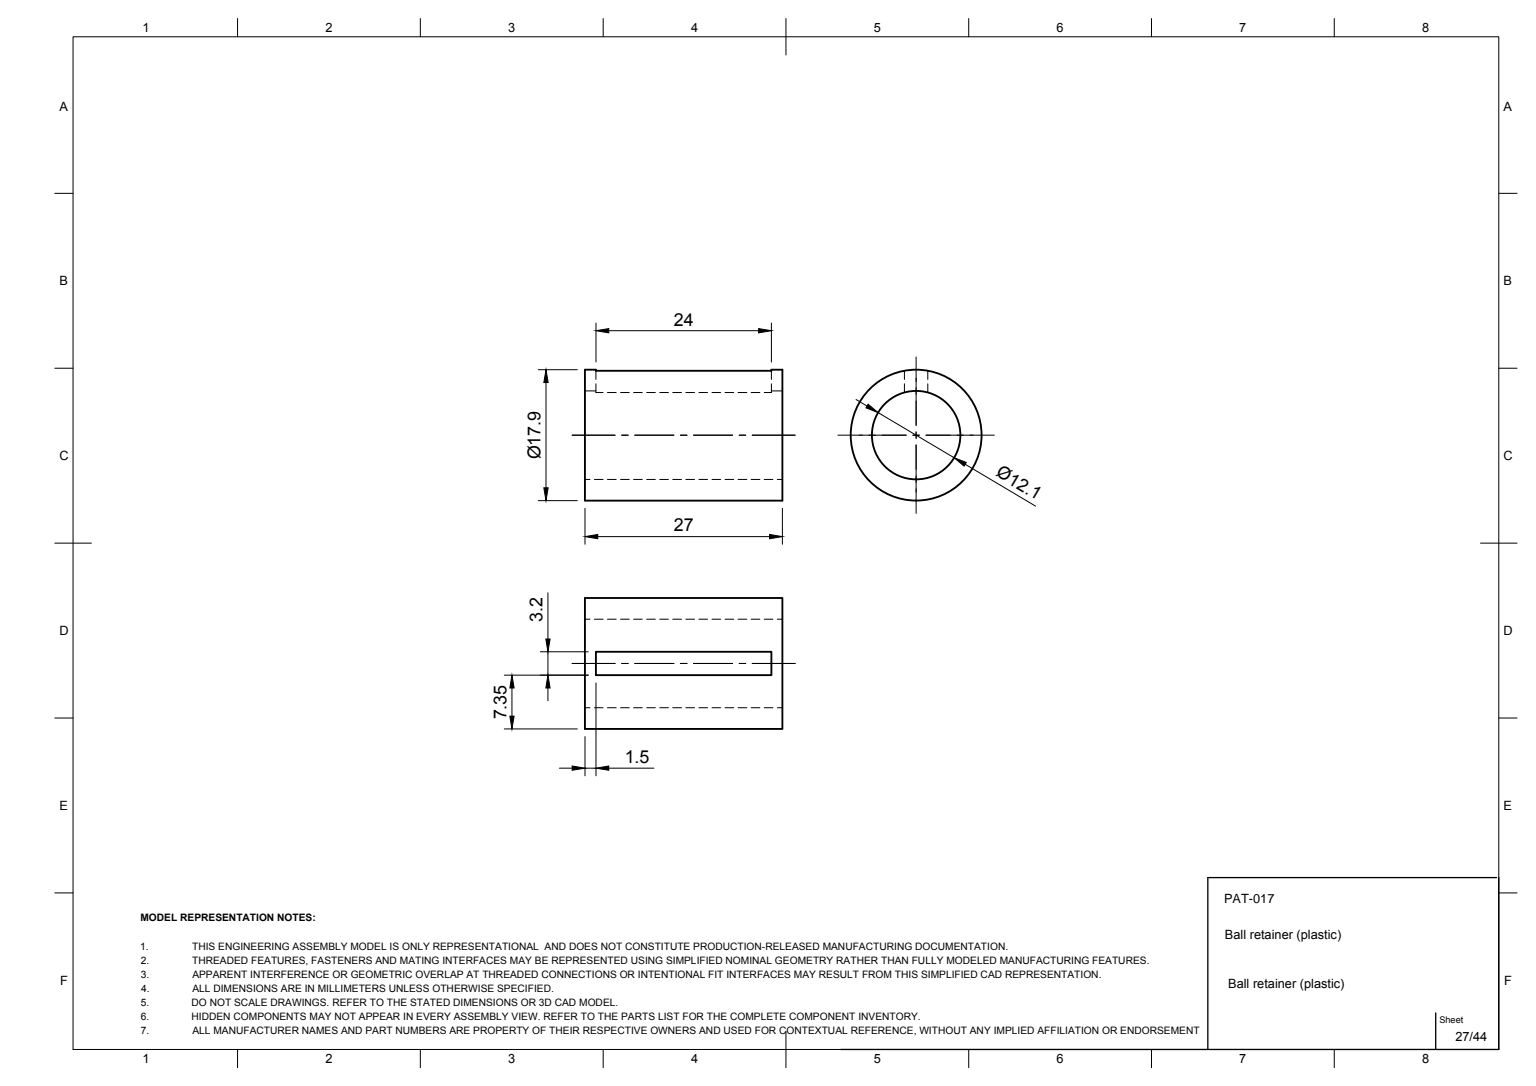
ISO-10303-21;
HEADER;
/* Generated by software containing ST-Developer
 * from STEP Tools, Inc. (www.steptools.com) 
 */

FILE_DESCRIPTION(
/* description */ ('Cam-and-follower valve demonstrator'),
/* implementation_level */ '2;1');

FILE_NAME(
/* name */ 'Ball retainer (plastic).step',
/* time_stamp */ '2026-10-28T03:25:17-07:00',
/* author */ (''),
/* organization */ (''),
/* preprocessor_version */ 'ST-DEVELOPER v20.2',
/* originating_system */ 'Autodesk Translation Framework v15.17.0.0',
/* authorisation */ '');

FILE_SCHEMA (('AUTOMOTIVE_DESIGN { 1 0 10303 214 3 1 1 }'));
ENDSEC;

DATA;
#10=MECHANICAL_DESIGN_GEOMETRIC_PRESENTATION_REPRESENTATION('',(#438),#12896);
#359=SHAPE_REPRESENTATION_RELATIONSHIP('SRR','None',#13077,#395);
#395=ADVANCED_BREP_SHAPE_REPRESENTATION('',(#480),#12877);
#438=STYLED_ITEM('',(#13323),#480);
#480=MANIFOLD_SOLID_BREP('Body1',#6206);
#621=FACE_BOUND('',#1823,.T.);
#622=FACE_BOUND('',#1825,.T.);
#623=FACE_BOUND('',#1827,.T.);
#624=FACE_BOUND('',#1829,.T.);
#882=CIRCLE('',#7103,0.895);
#883=CIRCLE('',#7104,0.605);
#884=CIRCLE('',#7107,0.895);
#885=CIRCLE('',#7108,0.605);
#886=CIRCLE('',#7111,0.895);
#887=CIRCLE('',#7112,0.605);
#888=CIRCLE('',#7114,0.895);
#889=CIRCLE('',#7116,0.605);
#1058=CYLINDRICAL_SURFACE('',#7113,0.895);
#1059=CYLINDRICAL_SURFACE('',#7117,0.605);
#1324=FACE_OUTER_BOUND('',#1818,.T.);
#1325=FACE_OUTER_BOUND('',#1819,.T.);
#1326=FACE_OUTER_BOUND('',#1820,.T.);
#1327=FACE_OUTER_BOUND('',#1821,.T.);
#1328=FACE_OUTER_BOUND('',#1822,.T.);
#1329=FACE_OUTER_BOUND('',#1824,.T.);
#1330=FACE_OUTER_BOUND('',#1826,.T.);
#1331=FACE_OUTER_BOUND('',#1828,.T.);
#1818=EDGE_LOOP('',(#5077,#5078,#5079,#5080));
#1819=EDGE_LOOP('',(#5081,#5082,#5083,#5084));
#1820=EDGE_LOOP('',(#5085,#5086,#5087,#5088));
#1821=EDGE_LOOP('',(#5089,#5090,#5091,#5092));
#1822=EDGE_LOOP('',(#5093));
#1823=EDGE_LOOP('',(#5094));
#1824=EDGE_LOOP('',(#5095,#5096,#5097,#5098));
#1825=EDGE_LOOP('',(#5099,#5100,#5101,#5102));
#1826=EDGE_LOOP('',(#5103));
#1827=EDGE_LOOP('',(#5104));
#1828=EDGE_LOOP('',(#5105,#5106,#5107,#5108));
#1829=EDGE_LOOP('',(#5109,#5110,#5111,#5112));
#2248=LINE('',#12164,#2670);
#2249=LINE('',#12167,#2671);
#2250=LINE('',#12170,#2672);
#2251=LINE('',#12172,#2673);
#2252=LINE('',#12173,#2674);
#2253=LINE('',#12179,#2675);
#2254=LINE('',#12181,#2676);
#2255=LINE('',#12182,#2677);
#2256=LINE('',#12191,#2678);
#2257=LINE('',#12196,#2679);
#2670=VECTOR('',#8631,1.);
#2671=VECTOR('',#8634,1.);
#2672=VECTOR('',#8637,1.);
#2673=VECTOR('',#8638,1.);
#2674=VECTOR('',#8639,1.);
#2675=VECTOR('',#8646,1.);
#2676=VECTOR('',#8649,1.);
#2677=VECTOR('',#8650,1.);
#2678=VECTOR('',#8661,0.895);
#2679=VECTOR('',#8668,0.605);
#3173=VERTEX_POINT('',#12160);
#3174=VERTEX_POINT('',#12161);
#3175=VERTEX_POINT('',#12163);
#3176=VERTEX_POINT('',#12165);
#3177=VERTEX_POINT('',#12169);
#3178=VERTEX_POINT('',#12171);
#3179=VERTEX_POINT('',#12175);
#3180=VERTEX_POINT('',#12177);
#3181=VERTEX_POINT('',#12184);
#3182=VERTEX_POINT('',#12186);
#3183=VERTEX_POINT('',#12189);
#3184=VERTEX_POINT('',#12193);
#3835=EDGE_CURVE('',#3173,#3174,#882,.T.);
#3836=EDGE_CURVE('',#3175,#3173,#2248,.T.);
#3837=EDGE_CURVE('',#3176,#3175,#883,.T.);
#3838=EDGE_CURVE('',#3174,#3176,#2249,.T.);
#3839=EDGE_CURVE('',#3174,#3177,#2250,.T.);
#3840=EDGE_CURVE('',#3178,#3176,#2251,.T.);
#3841=EDGE_CURVE('',#3178,#3177,#2252,.T.);
#3842=EDGE_CURVE('',#3177,#3179,#884,.T.);
#3843=EDGE_CURVE('',#3180,#3178,#885,.T.);
#3844=EDGE_CURVE('',#3179,#3180,#2253,.T.);
#3845=EDGE_CURVE('',#3179,#3173,#2254,.T.);
#3846=EDGE_CURVE('',#3175,#3180,#2255,.T.);
#3847=EDGE_CURVE('',#3181,#3181,#886,.T.);
#3848=EDGE_CURVE('',#3182,#3182,#887,.T.);
#3849=EDGE_CURVE('',#3183,#3183,#888,.T.);
#3850=EDGE_CURVE('',#3183,#3181,#2256,.T.);
#3851=EDGE_CURVE('',#3184,#3184,#889,.T.);
#3852=EDGE_CURVE('',#3184,#3182,#2257,.T.);
#5077=ORIENTED_EDGE('',*,*,#3835,.F.);
#5078=ORIENTED_EDGE('',*,*,#3836,.F.);
#5079=ORIENTED_EDGE('',*,*,#3837,.F.);
#5080=ORIENTED_EDGE('',*,*,#3838,.F.);
#5081=ORIENTED_EDGE('',*,*,#3839,.F.);
#5082=ORIENTED_EDGE('',*,*,#3838,.T.);
#5083=ORIENTED_EDGE('',*,*,#3840,.F.);
#5084=ORIENTED_EDGE('',*,*,#3841,.T.);
#5085=ORIENTED_EDGE('',*,*,#3842,.F.);
#5086=ORIENTED_EDGE('',*,*,#3841,.F.);
#5087=ORIENTED_EDGE('',*,*,#3843,.F.);
#5088=ORIENTED_EDGE('',*,*,#3844,.F.);
#5089=ORIENTED_EDGE('',*,*,#3845,.F.);
#5090=ORIENTED_EDGE('',*,*,#3844,.T.);
#5091=ORIENTED_EDGE('',*,*,#3846,.F.);
#5092=ORIENTED_EDGE('',*,*,#3836,.T.);
#5093=ORIENTED_EDGE('',*,*,#3847,.F.);
#5094=ORIENTED_EDGE('',*,*,#3848,.T.);
#5095=ORIENTED_EDGE('',*,*,#3849,.F.);
#5096=ORIENTED_EDGE('',*,*,#3850,.T.);
#5097=ORIENTED_EDGE('',*,*,#3847,.T.);
#5098=ORIENTED_EDGE('',*,*,#3850,.F.);
#5099=ORIENTED_EDGE('',*,*,#3842,.T.);
#5100=ORIENTED_EDGE('',*,*,#3845,.T.);
#5101=ORIENTED_EDGE('',*,*,#3835,.T.);
#5102=ORIENTED_EDGE('',*,*,#3839,.T.);
#5103=ORIENTED_EDGE('',*,*,#3849,.T.);
#5104=ORIENTED_EDGE('',*,*,#3851,.F.);
#5105=ORIENTED_EDGE('',*,*,#3851,.T.);
#5106=ORIENTED_EDGE('',*,*,#3852,.T.);
#5107=ORIENTED_EDGE('',*,*,#3848,.F.);
#5108=ORIENTED_EDGE('',*,*,#3852,.F.);
#5109=ORIENTED_EDGE('',*,*,#3843,.T.);
#5110=ORIENTED_EDGE('',*,*,#3840,.T.);
#5111=ORIENTED_EDGE('',*,*,#3837,.T.);
#5112=ORIENTED_EDGE('',*,*,#3846,.T.);
#5716=PLANE('',#7102);
#5717=PLANE('',#7105);
#5718=PLANE('',#7106);
#5719=PLANE('',#7109);
#5720=PLANE('',#7110);
#5721=PLANE('',#7115);
#6040=ADVANCED_FACE('',(#1324),#5716,.F.);
#6041=ADVANCED_FACE('',(#1325),#5717,.F.);
#6042=ADVANCED_FACE('',(#1326),#5718,.F.);
#6043=ADVANCED_FACE('',(#1327),#5719,.F.);
#6044=ADVANCED_FACE('',(#1328,#621),#5720,.T.);
#6045=ADVANCED_FACE('',(#1329,#622),#1058,.T.);
#6046=ADVANCED_FACE('',(#1330,#623),#5721,.T.);
#6047=ADVANCED_FACE('',(#1331,#624),#1059,.F.);
#6206=CLOSED_SHELL('',(#6040,#6041,#6042,#6043,#6044,#6045,#6046,#6047));
#7101=AXIS2_PLACEMENT_3D('',#12158,#8625,#8626);
#7102=AXIS2_PLACEMENT_3D('',#12159,#8627,#8628);
#7103=AXIS2_PLACEMENT_3D('',#12162,#8629,#8630);
#7104=AXIS2_PLACEMENT_3D('',#12166,#8632,#8633);
#7105=AXIS2_PLACEMENT_3D('',#12168,#8635,#8636);
#7106=AXIS2_PLACEMENT_3D('',#12174,#8640,#8641);
#7107=AXIS2_PLACEMENT_3D('',#12176,#8642,#8643);
#7108=AXIS2_PLACEMENT_3D('',#12178,#8644,#8645);
#7109=AXIS2_PLACEMENT_3D('',#12180,#8647,#8648);
#7110=AXIS2_PLACEMENT_3D('',#12183,#8651,#8652);
#7111=AXIS2_PLACEMENT_3D('',#12185,#8653,#8654);
#7112=AXIS2_PLACEMENT_3D('',#12187,#8655,#8656);
#7113=AXIS2_PLACEMENT_3D('',#12188,#8657,#8658);
#7114=AXIS2_PLACEMENT_3D('',#12190,#8659,#8660);
#7115=AXIS2_PLACEMENT_3D('',#12192,#8662,#8663);
#7116=AXIS2_PLACEMENT_3D('',#12194,#8664,#8665);
#7117=AXIS2_PLACEMENT_3D('',#12195,#8666,#8667);
#8625=DIRECTION('axis',(0.,0.,1.));
#8626=DIRECTION('refdir',(1.,0.,0.));
#8627=DIRECTION('center_axis',(0.,1.,0.));
#8628=DIRECTION('ref_axis',(0.,0.,1.));
#8629=DIRECTION('center_axis',(0.,1.,0.));
#8630=DIRECTION('ref_axis',(1.,0.,0.));
#8631=DIRECTION('',(1.,0.,0.));
#8632=DIRECTION('center_axis',(0.,-1.,0.));
#8633=DIRECTION('ref_axis',(1.,0.,0.));
#8634=DIRECTION('',(-1.,0.,0.));
#8635=DIRECTION('center_axis',(0.,0.,-1.));
#8636=DIRECTION('ref_axis',(-1.,0.,0.));
#8637=DIRECTION('',(0.,-1.,0.));
#8638=DIRECTION('',(0.,1.,0.));
#8639=DIRECTION('',(1.,0.,0.));
#8640=DIRECTION('center_axis',(0.,-1.,0.));
#8641=DIRECTION('ref_axis',(0.,0.,-1.));
#8642=DIRECTION('center_axis',(0.,-1.,0.));
#8643=DIRECTION('ref_axis',(1.,0.,0.));
#8644=DIRECTION('center_axis',(0.,1.,0.));
#8645=DIRECTION('ref_axis',(1.,0.,0.));
#8646=DIRECTION('',(-1.,0.,0.));
#8647=DIRECTION('center_axis',(0.,0.,1.));
#8648=DIRECTION('ref_axis',(1.,0.,0.));
#8649=DIRECTION('',(0.,1.,0.));
#8650=DIRECTION('',(0.,-1.,0.));
#8651=DIRECTION('center_axis',(0.,1.,0.));
#8652=DIRECTION('ref_axis',(0.,0.,1.));
#8653=DIRECTION('center_axis',(0.,-1.,0.));
#8654=DIRECTION('ref_axis',(1.,0.,0.));
#8655=DIRECTION('center_axis',(0.,-1.,0.));
#8656=DIRECTION('ref_axis',(1.,0.,0.));
#8657=DIRECTION('center_axis',(0.,-1.,0.));
#8658=DIRECTION('ref_axis',(1.,0.,0.));
#8659=DIRECTION('center_axis',(0.,-1.,0.));
#8660=DIRECTION('ref_axis',(1.,0.,0.));
#8661=DIRECTION('',(0.,1.,0.));
#8662=DIRECTION('center_axis',(0.,-1.,0.));
#8663=DIRECTION('ref_axis',(0.,0.,-1.));
#8664=DIRECTION('center_axis',(0.,-1.,0.));
#8665=DIRECTION('ref_axis',(1.,0.,0.));
#8666=DIRECTION('center_axis',(0.,-1.,0.));
#8667=DIRECTION('ref_axis',(1.,0.,0.));
#8668=DIRECTION('',(0.,1.,0.));
#12158=CARTESIAN_POINT('',(0.,0.,0.));
#12159=CARTESIAN_POINT('Origin',(0.75,1.2,0.));
#12160=CARTESIAN_POINT('',(0.880582193778639,1.2,0.16));
#12161=CARTESIAN_POINT('',(0.880582193778639,1.2,-0.16));
#12162=CARTESIAN_POINT('Origin',(0.,1.2,0.));
#12163=CARTESIAN_POINT('',(0.583459510163302,1.2,0.16));
#12164=CARTESIAN_POINT('',(0.57,1.2,0.16));
#12165=CARTESIAN_POINT('',(0.583459510163302,1.2,-0.16));
#12166=CARTESIAN_POINT('Origin',(0.,1.2,0.));
#12167=CARTESIAN_POINT('',(0.93,1.2,-0.16));
#12168=CARTESIAN_POINT('Origin',(0.93,0.,-0.16));
#12169=CARTESIAN_POINT('',(0.880582193778639,-1.2,-0.16));
#12170=CARTESIAN_POINT('',(0.880582193778639,0.,-0.16));
#12171=CARTESIAN_POINT('',(0.583459510163302,-1.2,-0.16));
#12172=CARTESIAN_POINT('',(0.583459510163302,0.,-0.16));
#12173=CARTESIAN_POINT('',(0.93,-1.2,-0.16));
#12174=CARTESIAN_POINT('Origin',(0.75,-1.2,0.));
#12175=CARTESIAN_POINT('',(0.880582193778639,-1.2,0.16));
#12176=CARTESIAN_POINT('Origin',(0.,-1.2,0.));
#12177=CARTESIAN_POINT('',(0.583459510163302,-1.2,0.16));
#12178=CARTESIAN_POINT('Origin',(0.,-1.2,0.));
#12179=CARTESIAN_POINT('',(0.57,-1.2,0.16));
#12180=CARTESIAN_POINT('Origin',(0.57,0.,0.16));
#12181=CARTESIAN_POINT('',(0.880582193778639,0.,0.16));
#12182=CARTESIAN_POINT('',(0.583459510163302,0.,0.16));
#12183=CARTESIAN_POINT('Origin',(0.895,1.35,0.));
#12184=CARTESIAN_POINT('',(-0.895,1.35,-1.09605888523688E-16));
#12185=CARTESIAN_POINT('Origin',(0.,1.35,0.));
#12186=CARTESIAN_POINT('',(-0.605,1.35,-7.40911313484149E-17));
#12187=CARTESIAN_POINT('Origin',(0.,1.35,0.));
#12188=CARTESIAN_POINT('Origin',(0.,0.,0.));
#12189=CARTESIAN_POINT('',(-0.895,-1.35,-1.09605888523688E-16));
#12190=CARTESIAN_POINT('Origin',(0.,-1.35,0.));
#12191=CARTESIAN_POINT('',(-0.895,0.,-1.09605888523688E-16));
#12192=CARTESIAN_POINT('Origin',(0.605,-1.35,0.));
#12193=CARTESIAN_POINT('',(-0.605,-1.35,-7.40911313484149E-17));
#12194=CARTESIAN_POINT('Origin',(0.,-1.35,0.));
#12195=CARTESIAN_POINT('Origin',(0.,0.,0.));
#12196=CARTESIAN_POINT('',(-0.605,0.,-7.40911313484149E-17));
#12834=UNCERTAINTY_MEASURE_WITH_UNIT(LENGTH_MEASURE(0.001),#12897,
'DISTANCE_ACCURACY_VALUE',
'Maximum model space distance between geometric entities at asserted c
onnectivities');
#12853=UNCERTAINTY_MEASURE_WITH_UNIT(LENGTH_MEASURE(0.001),#12897,
'DISTANCE_ACCURACY_VALUE',
'Maximum model space distance between geometric entities at asserted c
onnectivities');
#12877=(
GEOMETRIC_REPRESENTATION_CONTEXT(3)
GLOBAL_UNCERTAINTY_ASSIGNED_CONTEXT((#12834))
GLOBAL_UNIT_ASSIGNED_CONTEXT((#12897,#12899,#12900))
REPRESENTATION_CONTEXT('','3D')
);
#12896=(
GEOMETRIC_REPRESENTATION_CONTEXT(3)
GLOBAL_UNCERTAINTY_ASSIGNED_CONTEXT((#12853))
GLOBAL_UNIT_ASSIGNED_CONTEXT((#12897,#12899,#12900))
REPRESENTATION_CONTEXT('','3D')
);
#12897=(
LENGTH_UNIT()
NAMED_UNIT(*)
SI_UNIT(.CENTI.,.METRE.)
);
#12899=(
NAMED_UNIT(*)
PLANE_ANGLE_UNIT()
SI_UNIT($,.RADIAN.)
);
#12900=(
NAMED_UNIT(*)
SI_UNIT($,.STERADIAN.)
SOLID_ANGLE_UNIT()
);
#12924=SHAPE_DEFINITION_REPRESENTATION(#12971,#13077);
#12971=PRODUCT_DEFINITION_SHAPE('',$,#13120);
#13077=SHAPE_REPRESENTATION('',(#7101),#12877);
#13096=PRODUCT_DEFINITION_CONTEXT('part definition',#13224,'design');
#13120=PRODUCT_DEFINITION('Ball retainer (plastic)',
'Ball retainer (plastic)',#13162,#13096);
#13162=PRODUCT_DEFINITION_FORMATION('',$,#13249);
#13224=APPLICATION_CONTEXT(
'Core Data for Automotive Mechanical Design Process');
#13225=PRODUCT_CONTEXT('part definition',#13224,'mechanical');
#13249=PRODUCT('Ball retainer (plastic)','Ball retainer (plastic)',
'Ball retainer (plastic)',(#13225));
#13317=COLOUR_RGB('Sky Blue',0.24,0.69,0.87);
#13318=FILL_AREA_STYLE_COLOUR('',#13317);
#13319=FILL_AREA_STYLE('',(#13318));
#13320=SURFACE_STYLE_FILL_AREA(#13319);
#13321=SURFACE_SIDE_STYLE('',(#13320));
#13322=SURFACE_STYLE_USAGE(.BOTH.,#13321);
#13323=PRESENTATION_STYLE_ASSIGNMENT((#13322));
ENDSEC;
END-ISO-10303-21;
